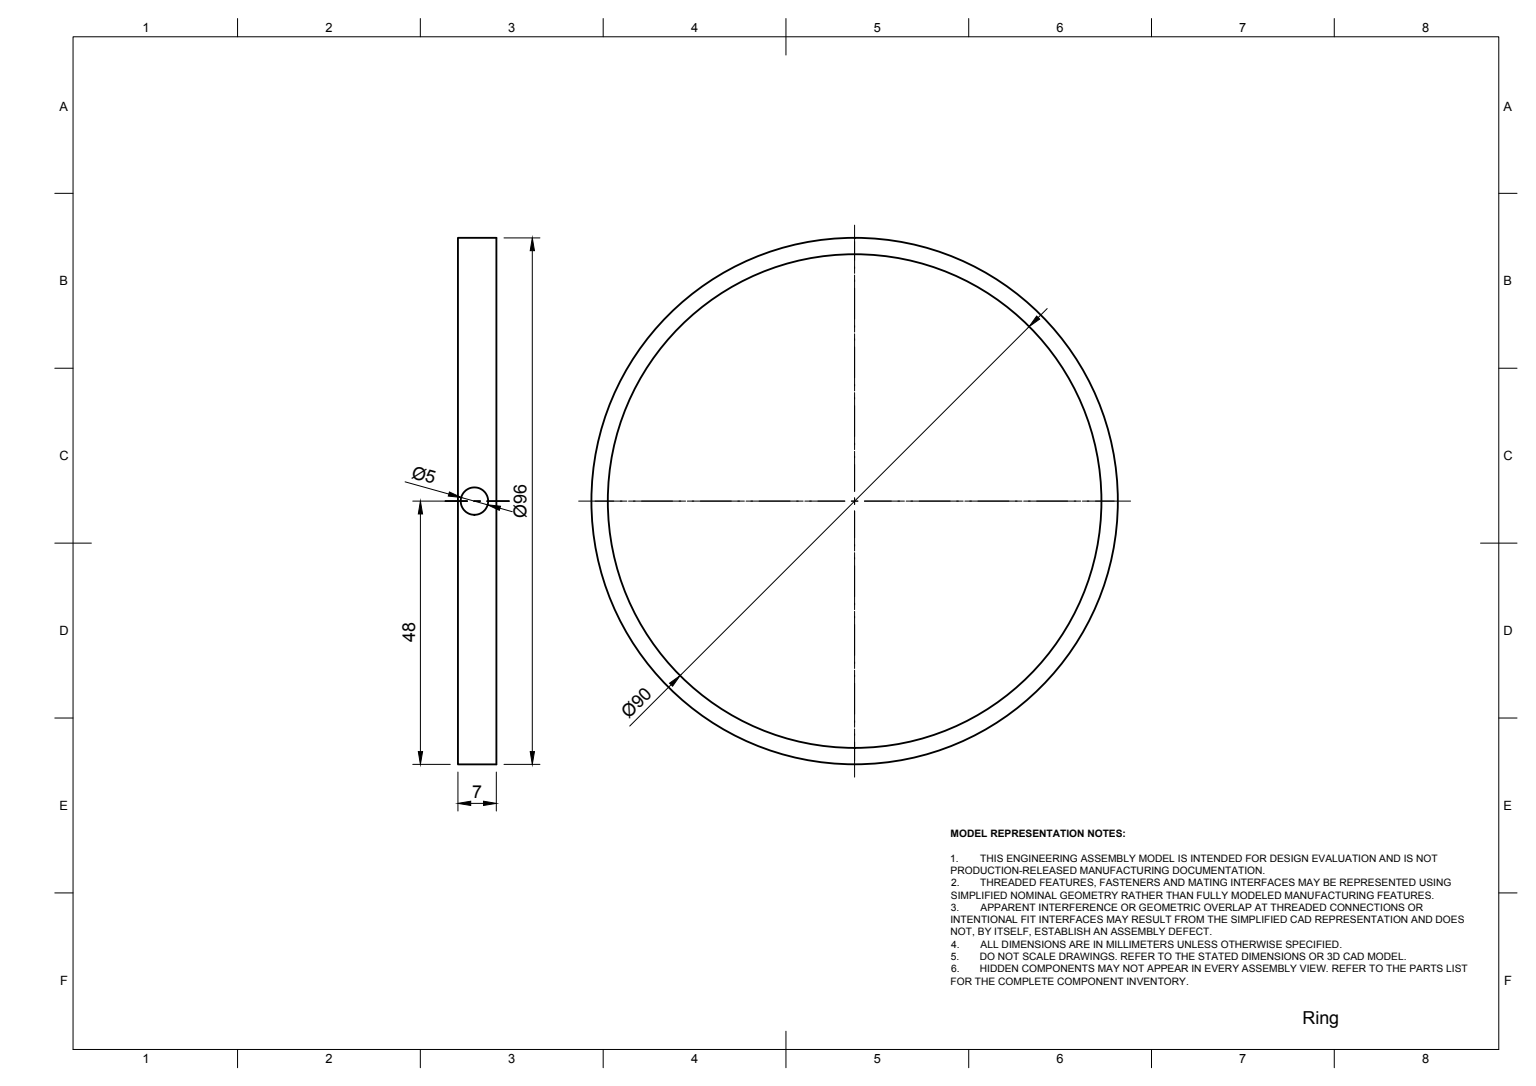
ISO-10303-21;
HEADER;
/* Generated by software containing ST-Developer
 * from STEP Tools, Inc. (www.steptools.com) 
 */

FILE_DESCRIPTION(
/* description */ (''),
/* implementation_level */ '2;1');

FILE_NAME(
/* name */ 'Ring.step',
/* time_stamp */ '2026-10-04T12:17:52-07:00',
/* author */ (''),
/* organization */ (''),
/* preprocessor_version */ 'ST-DEVELOPER v20.2',
/* originating_system */ 'Autodesk Translation Framework v15.15.0.0',
/* authorisation */ '');

FILE_SCHEMA (('AUTOMOTIVE_DESIGN { 1 0 10303 214 3 1 1 }'));
ENDSEC;

DATA;
#10=MECHANICAL_DESIGN_GEOMETRIC_PRESENTATION_REPRESENTATION('',(#65),#1602);
#43=B_SPLINE_CURVE_WITH_KNOTS('',3,(#1356,#1357,#1358,#1359,#1360,#1361,
#1362,#1363,#1364,#1365,#1366,#1367,#1368,#1369,#1370,#1371,#1372,#1373,
#1374,#1375,#1376,#1377,#1378,#1379,#1380,#1381,#1382,#1383,#1384,#1385,
#1386,#1387,#1388,#1389),.UNSPECIFIED.,.T.,.F.,(4,2,2,2,2,2,2,2,2,2,2,2,
2,2,2,2,4),(0.,0.0941899649900925,0.188379929980185,0.282569871539204,0.376759813098223,
0.470949754657242,0.565139696216261,0.659329661206353,0.753519626196446,
0.847709591186538,0.941899556176631,1.03608949773565,1.13027943929467,1.22446938085369,
1.31865932241271,1.4128492874028,1.50703925239289),.UNSPECIFIED.);
#44=B_SPLINE_CURVE_WITH_KNOTS('',3,(#1392,#1393,#1394,#1395,#1396,#1397,
#1398,#1399,#1400,#1401,#1402,#1403,#1404,#1405,#1406,#1407,#1408,#1409,
#1410,#1411,#1412,#1413,#1414,#1415,#1416,#1417,#1418,#1419,#1420,#1421,
#1422,#1423,#1424,#1425),.UNSPECIFIED.,.T.,.F.,(4,2,2,2,2,2,2,2,2,2,2,2,
2,2,2,2,4),(-1.50707960704781,-1.41288711643541,-1.318694625823,-1.22450216555443,
-1.13030970528586,-1.03611724501729,-0.941924784748718,-0.847732294136312,
-0.753539803523906,-0.6593473129115,-0.565154822299094,-0.470962362030524,
-0.376769901761953,-0.282577441493383,-0.188384981224812,-0.094192490612406,
0.),.UNSPECIFIED.);
#45=B_SPLINE_CURVE_WITH_KNOTS('',3,(#1428,#1429,#1430,#1431,#1432,#1433,
#1434,#1435,#1436,#1437,#1438,#1439,#1440,#1441,#1442,#1443,#1444,#1445,
#1446,#1447,#1448,#1449,#1450,#1451,#1452,#1453,#1454,#1455,#1456,#1457,
#1458,#1459,#1460,#1461),.UNSPECIFIED.,.T.,.F.,(4,2,2,2,2,2,2,2,2,2,2,2,
2,2,2,2,4),(-1.50707960704781,-1.41288711643541,-1.318694625823,-1.22450216555443,
-1.13030970528586,-1.03611724501729,-0.941924784748719,-0.847732294136313,
-0.753539803523906,-0.6593473129115,-0.565154822299094,-0.470962362030524,
-0.376769901761953,-0.282577441493383,-0.188384981224812,-0.0941924906124062,
0.),.UNSPECIFIED.);
#46=B_SPLINE_CURVE_WITH_KNOTS('',3,(#1464,#1465,#1466,#1467,#1468,#1469,
#1470,#1471,#1472,#1473,#1474,#1475,#1476,#1477,#1478,#1479,#1480,#1481,
#1482,#1483,#1484,#1485,#1486,#1487,#1488,#1489,#1490,#1491,#1492,#1493,
#1494,#1495,#1496,#1497),.UNSPECIFIED.,.T.,.F.,(4,2,2,2,2,2,2,2,2,2,2,2,
2,2,2,2,4),(0.,0.0941899649900927,0.188379929980185,0.282569871539204,0.376759813098223,
0.470949754657242,0.565139696216261,0.659329661206353,0.753519626196446,
0.847709591186538,0.941899556176631,1.03608949773565,1.13027943929467,1.22446938085369,
1.31865932241271,1.4128492874028,1.50703925239289),.UNSPECIFIED.);
#49=SHAPE_REPRESENTATION_RELATIONSHIP('SRR','None',#1636,#57);
#57=ADVANCED_BREP_SHAPE_REPRESENTATION('',(#73),#1596);
#65=STYLED_ITEM('',(#1684),#73);
#73=MANIFOLD_SOLID_BREP('Body1',#776);
#81=FACE_BOUND('',#230,.T.);
#82=FACE_BOUND('',#231,.T.);
#83=FACE_BOUND('',#233,.T.);
#84=FACE_BOUND('',#234,.T.);
#85=FACE_BOUND('',#236,.T.);
#86=FACE_BOUND('',#238,.T.);
#113=CIRCLE('',#921,45.);
#114=CIRCLE('',#922,45.);
#115=CIRCLE('',#924,48.);
#116=CIRCLE('',#925,48.);
#143=CYLINDRICAL_SURFACE('',#918,2.5);
#144=CYLINDRICAL_SURFACE('',#919,2.5);
#145=CYLINDRICAL_SURFACE('',#920,45.);
#146=CYLINDRICAL_SURFACE('',#923,48.);
#178=FACE_OUTER_BOUND('',#227,.T.);
#179=FACE_OUTER_BOUND('',#228,.T.);
#180=FACE_OUTER_BOUND('',#229,.T.);
#181=FACE_OUTER_BOUND('',#232,.T.);
#182=FACE_OUTER_BOUND('',#235,.T.);
#183=FACE_OUTER_BOUND('',#237,.T.);
#227=EDGE_LOOP('',(#630,#631,#632,#633));
#228=EDGE_LOOP('',(#634,#635,#636,#637));
#229=EDGE_LOOP('',(#638,#639,#640,#641));
#230=EDGE_LOOP('',(#642));
#231=EDGE_LOOP('',(#643));
#232=EDGE_LOOP('',(#644,#645,#646,#647));
#233=EDGE_LOOP('',(#648));
#234=EDGE_LOOP('',(#649));
#235=EDGE_LOOP('',(#650));
#236=EDGE_LOOP('',(#651));
#237=EDGE_LOOP('',(#652));
#238=EDGE_LOOP('',(#653));
#300=LINE('',#1391,#349);
#301=LINE('',#1463,#350);
#302=LINE('',#1502,#351);
#303=LINE('',#1508,#352);
#349=VECTOR('',#1108,2.5);
#350=VECTOR('',#1111,2.5);
#351=VECTOR('',#1116,45.);
#352=VECTOR('',#1123,48.);
#399=VERTEX_POINT('',#1355);
#400=VERTEX_POINT('',#1390);
#401=VERTEX_POINT('',#1427);
#402=VERTEX_POINT('',#1462);
#403=VERTEX_POINT('',#1499);
#404=VERTEX_POINT('',#1501);
#405=VERTEX_POINT('',#1505);
#406=VERTEX_POINT('',#1507);
#480=EDGE_CURVE('',#399,#399,#43,.T.);
#481=EDGE_CURVE('',#399,#400,#300,.T.);
#482=EDGE_CURVE('',#400,#400,#44,.T.);
#483=EDGE_CURVE('',#401,#401,#45,.T.);
#484=EDGE_CURVE('',#401,#402,#301,.T.);
#485=EDGE_CURVE('',#402,#402,#46,.T.);
#486=EDGE_CURVE('',#403,#403,#113,.T.);
#487=EDGE_CURVE('',#403,#404,#302,.T.);
#488=EDGE_CURVE('',#404,#404,#114,.T.);
#489=EDGE_CURVE('',#405,#405,#115,.T.);
#490=EDGE_CURVE('',#405,#406,#303,.T.);
#491=EDGE_CURVE('',#406,#406,#116,.T.);
#630=ORIENTED_EDGE('',*,*,#480,.F.);
#631=ORIENTED_EDGE('',*,*,#481,.T.);
#632=ORIENTED_EDGE('',*,*,#482,.F.);
#633=ORIENTED_EDGE('',*,*,#481,.F.);
#634=ORIENTED_EDGE('',*,*,#483,.F.);
#635=ORIENTED_EDGE('',*,*,#484,.T.);
#636=ORIENTED_EDGE('',*,*,#485,.F.);
#637=ORIENTED_EDGE('',*,*,#484,.F.);
#638=ORIENTED_EDGE('',*,*,#486,.T.);
#639=ORIENTED_EDGE('',*,*,#487,.T.);
#640=ORIENTED_EDGE('',*,*,#488,.F.);
#641=ORIENTED_EDGE('',*,*,#487,.F.);
#642=ORIENTED_EDGE('',*,*,#482,.T.);
#643=ORIENTED_EDGE('',*,*,#483,.T.);
#644=ORIENTED_EDGE('',*,*,#489,.F.);
#645=ORIENTED_EDGE('',*,*,#490,.T.);
#646=ORIENTED_EDGE('',*,*,#491,.T.);
#647=ORIENTED_EDGE('',*,*,#490,.F.);
#648=ORIENTED_EDGE('',*,*,#480,.T.);
#649=ORIENTED_EDGE('',*,*,#485,.T.);
#650=ORIENTED_EDGE('',*,*,#489,.T.);
#651=ORIENTED_EDGE('',*,*,#488,.T.);
#652=ORIENTED_EDGE('',*,*,#491,.F.);
#653=ORIENTED_EDGE('',*,*,#486,.F.);
#715=PLANE('',#926);
#716=PLANE('',#927);
#750=ADVANCED_FACE('',(#178),#143,.F.);
#751=ADVANCED_FACE('',(#179),#144,.F.);
#752=ADVANCED_FACE('',(#180,#81,#82),#145,.F.);
#753=ADVANCED_FACE('',(#181,#83,#84),#146,.T.);
#754=ADVANCED_FACE('',(#182,#85),#715,.T.);
#755=ADVANCED_FACE('',(#183,#86),#716,.F.);
#776=CLOSED_SHELL('',(#750,#751,#752,#753,#754,#755));
#917=AXIS2_PLACEMENT_3D('',#1353,#1104,#1105);
#918=AXIS2_PLACEMENT_3D('',#1354,#1106,#1107);
#919=AXIS2_PLACEMENT_3D('',#1426,#1109,#1110);
#920=AXIS2_PLACEMENT_3D('',#1498,#1112,#1113);
#921=AXIS2_PLACEMENT_3D('',#1500,#1114,#1115);
#922=AXIS2_PLACEMENT_3D('',#1503,#1117,#1118);
#923=AXIS2_PLACEMENT_3D('',#1504,#1119,#1120);
#924=AXIS2_PLACEMENT_3D('',#1506,#1121,#1122);
#925=AXIS2_PLACEMENT_3D('',#1509,#1124,#1125);
#926=AXIS2_PLACEMENT_3D('',#1510,#1126,#1127);
#927=AXIS2_PLACEMENT_3D('',#1511,#1128,#1129);
#1104=DIRECTION('axis',(0.,0.,1.));
#1105=DIRECTION('refdir',(1.,0.,0.));
#1106=DIRECTION('center_axis',(0.,0.,1.));
#1107=DIRECTION('ref_axis',(1.,0.,0.));
#1108=DIRECTION('',(0.,0.,1.));
#1109=DIRECTION('center_axis',(0.,0.,1.));
#1110=DIRECTION('ref_axis',(1.,0.,0.));
#1111=DIRECTION('',(0.,0.,1.));
#1112=DIRECTION('center_axis',(0.,-1.,0.));
#1113=DIRECTION('ref_axis',(1.,0.,0.));
#1114=DIRECTION('center_axis',(0.,1.,0.));
#1115=DIRECTION('ref_axis',(1.,0.,0.));
#1116=DIRECTION('',(0.,-1.,0.));
#1117=DIRECTION('center_axis',(0.,1.,0.));
#1118=DIRECTION('ref_axis',(1.,0.,0.));
#1119=DIRECTION('center_axis',(0.,-1.,0.));
#1120=DIRECTION('ref_axis',(1.,0.,0.));
#1121=DIRECTION('center_axis',(0.,-1.,0.));
#1122=DIRECTION('ref_axis',(1.,0.,0.));
#1123=DIRECTION('',(0.,1.,0.));
#1124=DIRECTION('center_axis',(0.,-1.,0.));
#1125=DIRECTION('ref_axis',(1.,0.,0.));
#1126=DIRECTION('center_axis',(0.,-1.,0.));
#1127=DIRECTION('ref_axis',(1.,0.,0.));
#1128=DIRECTION('center_axis',(0.,-1.,0.));
#1129=DIRECTION('ref_axis',(1.,0.,0.));
#1353=CARTESIAN_POINT('',(0.,0.,0.));
#1354=CARTESIAN_POINT('Origin',(0.,0.,0.));
#1355=CARTESIAN_POINT('',(-2.5,-6.93889390390723E-17,2.06514837824155));
#1356=CARTESIAN_POINT('Ctrl Pts',(-2.5,0.,2.06514837824153));
#1357=CARTESIAN_POINT('Ctrl Pts',(-2.5,-0.313966549966975,2.06514837824153));
#1358=CARTESIAN_POINT('Ctrl Pts',(-2.43724208175823,-0.648821661237632,
2.06174633522331));
#1359=CARTESIAN_POINT('Ctrl Pts',(-2.18209026124743,-1.26475318832061,2.04945469062714));
#1360=CARTESIAN_POINT('Ctrl Pts',(-1.98969948627882,-1.54583441965392,2.04074211479646));
#1361=CARTESIAN_POINT('Ctrl Pts',(-1.54583447486274,-1.98969943106999,2.02438414468301));
#1362=CARTESIAN_POINT('Ctrl Pts',(-1.26475321841524,-2.18209024745813,2.0156767273781));
#1363=CARTESIAN_POINT('Ctrl Pts',(-0.648821611717717,-2.43724210359452,
2.00339687904366));
#1364=CARTESIAN_POINT('Ctrl Pts',(-0.313966471863397,-2.5,1.99999999999999));
#1365=CARTESIAN_POINT('Ctrl Pts',(0.313966471863396,-2.5,1.99999999999999));
#1366=CARTESIAN_POINT('Ctrl Pts',(0.648821611717716,-2.43724210359452,2.00339687904366));
#1367=CARTESIAN_POINT('Ctrl Pts',(1.26475321841524,-2.18209024745813,2.0156767273781));
#1368=CARTESIAN_POINT('Ctrl Pts',(1.54583447486274,-1.98969943106999,2.02438414468301));
#1369=CARTESIAN_POINT('Ctrl Pts',(1.98969948627882,-1.54583441965392,2.04074211479646));
#1370=CARTESIAN_POINT('Ctrl Pts',(2.18209026124743,-1.26475318832061,2.04945469062714));
#1371=CARTESIAN_POINT('Ctrl Pts',(2.43724208175823,-0.648821661237632,2.06174633522331));
#1372=CARTESIAN_POINT('Ctrl Pts',(2.5,-0.313966549966975,2.06514837824153));
#1373=CARTESIAN_POINT('Ctrl Pts',(2.5,0.313966549966975,2.06514837824153));
#1374=CARTESIAN_POINT('Ctrl Pts',(2.43724208175823,0.648821661237632,2.06174633522331));
#1375=CARTESIAN_POINT('Ctrl Pts',(2.18209026124743,1.26475318832061,2.04945469062714));
#1376=CARTESIAN_POINT('Ctrl Pts',(1.98969948627882,1.54583441965392,2.04074211479646));
#1377=CARTESIAN_POINT('Ctrl Pts',(1.54583447486274,1.98969943106999,2.02438414468301));
#1378=CARTESIAN_POINT('Ctrl Pts',(1.26475321841524,2.18209024745813,2.0156767273781));
#1379=CARTESIAN_POINT('Ctrl Pts',(0.648821611717718,2.43724210359452,2.00339687904366));
#1380=CARTESIAN_POINT('Ctrl Pts',(0.313966471863397,2.5,1.99999999999999));
#1381=CARTESIAN_POINT('Ctrl Pts',(-0.313966471863395,2.5,1.99999999999999));
#1382=CARTESIAN_POINT('Ctrl Pts',(-0.648821611717715,2.43724210359452,2.00339687904366));
#1383=CARTESIAN_POINT('Ctrl Pts',(-1.26475321841524,2.18209024745813,2.0156767273781));
#1384=CARTESIAN_POINT('Ctrl Pts',(-1.54583447486274,1.98969943107,2.02438414468301));
#1385=CARTESIAN_POINT('Ctrl Pts',(-1.98969948627882,1.54583441965392,2.04074211479646));
#1386=CARTESIAN_POINT('Ctrl Pts',(-2.18209026124743,1.26475318832061,2.04945469062714));
#1387=CARTESIAN_POINT('Ctrl Pts',(-2.43724208175823,0.648821661237633,2.06174633522331));
#1388=CARTESIAN_POINT('Ctrl Pts',(-2.5,0.313966549966975,2.06514837824153));
#1389=CARTESIAN_POINT('Ctrl Pts',(-2.5,-1.38777878078145E-16,2.06514837824153));
#1390=CARTESIAN_POINT('',(-2.5,-1.38777878078145E-16,5.06949811097144));
#1391=CARTESIAN_POINT('',(-2.5,-3.06161699786838E-16,0.));
#1392=CARTESIAN_POINT('Ctrl Pts',(-2.5,-2.08166817117217E-16,5.06949811097143));
#1393=CARTESIAN_POINT('Ctrl Pts',(-2.5,0.31397496870802,5.06949811097143));
#1394=CARTESIAN_POINT('Ctrl Pts',(-2.43723879407712,0.648833697924306,5.06586836285142));
#1395=CARTESIAN_POINT('Ctrl Pts',(-2.18208453863604,1.26476290215938,5.05275507922167));
#1396=CARTESIAN_POINT('Ctrl Pts',(-1.98969504628277,1.54583885964997,5.04346052213127));
#1397=CARTESIAN_POINT('Ctrl Pts',(-1.54583893114345,1.98969497478929,5.02601073765469));
#1398=CARTESIAN_POINT('Ctrl Pts',(-1.26476294130742,2.18208452114785,5.01672244237508));
#1399=CARTESIAN_POINT('Ctrl Pts',(-0.64883363366083,2.4372388219696,5.00362347878181));
#1400=CARTESIAN_POINT('Ctrl Pts',(-0.313974867561901,2.5,5.));
#1401=CARTESIAN_POINT('Ctrl Pts',(0.313974867561902,2.5,5.));
#1402=CARTESIAN_POINT('Ctrl Pts',(0.648833633660831,2.4372388219696,5.00362347878181));
#1403=CARTESIAN_POINT('Ctrl Pts',(1.26476294130743,2.18208452114784,5.01672244237508));
#1404=CARTESIAN_POINT('Ctrl Pts',(1.54583893114345,1.98969497478929,5.02601073765469));
#1405=CARTESIAN_POINT('Ctrl Pts',(1.98969504628277,1.54583885964996,5.04346052213127));
#1406=CARTESIAN_POINT('Ctrl Pts',(2.18208453863604,1.26476290215938,5.05275507922167));
#1407=CARTESIAN_POINT('Ctrl Pts',(2.43723879407712,0.648833697924305,5.06586836285142));
#1408=CARTESIAN_POINT('Ctrl Pts',(2.5,0.31397496870802,5.06949811097143));
#1409=CARTESIAN_POINT('Ctrl Pts',(2.5,-0.31397496870802,5.06949811097143));
#1410=CARTESIAN_POINT('Ctrl Pts',(2.43723879407712,-0.648833697924305,5.06586836285142));
#1411=CARTESIAN_POINT('Ctrl Pts',(2.18208453863604,-1.26476290215938,5.05275507922167));
#1412=CARTESIAN_POINT('Ctrl Pts',(1.98969504628277,-1.54583885964996,5.04346052213127));
#1413=CARTESIAN_POINT('Ctrl Pts',(1.54583893114345,-1.98969497478929,5.02601073765469));
#1414=CARTESIAN_POINT('Ctrl Pts',(1.26476294130743,-2.18208452114784,5.01672244237508));
#1415=CARTESIAN_POINT('Ctrl Pts',(0.648833633660831,-2.4372388219696,5.00362347878181));
#1416=CARTESIAN_POINT('Ctrl Pts',(0.313974867561901,-2.5,5.));
#1417=CARTESIAN_POINT('Ctrl Pts',(-0.313974867561902,-2.5,5.));
#1418=CARTESIAN_POINT('Ctrl Pts',(-0.648833633660832,-2.4372388219696,5.00362347878181));
#1419=CARTESIAN_POINT('Ctrl Pts',(-1.26476294130743,-2.18208452114784,5.01672244237508));
#1420=CARTESIAN_POINT('Ctrl Pts',(-1.54583893114345,-1.98969497478929,5.02601073765469));
#1421=CARTESIAN_POINT('Ctrl Pts',(-1.98969504628277,-1.54583885964996,5.04346052213127));
#1422=CARTESIAN_POINT('Ctrl Pts',(-2.18208453863604,-1.26476290215938,5.05275507922167));
#1423=CARTESIAN_POINT('Ctrl Pts',(-2.43723879407712,-0.648833697924305,
5.06586836285142));
#1424=CARTESIAN_POINT('Ctrl Pts',(-2.5,-0.31397496870802,5.06949811097143));
#1425=CARTESIAN_POINT('Ctrl Pts',(-2.5,6.93889390390723E-17,5.06949811097143));
#1426=CARTESIAN_POINT('Origin',(0.,0.,96.6));
#1427=CARTESIAN_POINT('',(-2.5,6.93889390390723E-17,94.9305018890286));
#1428=CARTESIAN_POINT('Ctrl Pts',(-2.5,1.38777878078145E-16,94.9305018890286));
#1429=CARTESIAN_POINT('Ctrl Pts',(-2.5,-0.31397496870802,94.9305018890286));
#1430=CARTESIAN_POINT('Ctrl Pts',(-2.43723879407712,-0.648833697924305,
94.9341316371486));
#1431=CARTESIAN_POINT('Ctrl Pts',(-2.18208453863604,-1.26476290215938,94.9472449207783));
#1432=CARTESIAN_POINT('Ctrl Pts',(-1.98969504628277,-1.54583885964996,94.9565394778687));
#1433=CARTESIAN_POINT('Ctrl Pts',(-1.54583893114345,-1.98969497478929,94.9739892623453));
#1434=CARTESIAN_POINT('Ctrl Pts',(-1.26476294130743,-2.18208452114784,94.9832775576249));
#1435=CARTESIAN_POINT('Ctrl Pts',(-0.648833633660833,-2.4372388219696,94.9963765212182));
#1436=CARTESIAN_POINT('Ctrl Pts',(-0.313974867561903,-2.5,95.));
#1437=CARTESIAN_POINT('Ctrl Pts',(0.313974867561902,-2.5,95.));
#1438=CARTESIAN_POINT('Ctrl Pts',(0.648833633660832,-2.4372388219696,94.9963765212182));
#1439=CARTESIAN_POINT('Ctrl Pts',(1.26476294130743,-2.18208452114784,94.9832775576249));
#1440=CARTESIAN_POINT('Ctrl Pts',(1.54583893114345,-1.98969497478929,94.9739892623453));
#1441=CARTESIAN_POINT('Ctrl Pts',(1.98969504628277,-1.54583885964996,94.9565394778687));
#1442=CARTESIAN_POINT('Ctrl Pts',(2.18208453863604,-1.26476290215938,94.9472449207783));
#1443=CARTESIAN_POINT('Ctrl Pts',(2.43723879407712,-0.648833697924305,94.9341316371486));
#1444=CARTESIAN_POINT('Ctrl Pts',(2.5,-0.31397496870802,94.9305018890286));
#1445=CARTESIAN_POINT('Ctrl Pts',(2.5,0.31397496870802,94.9305018890286));
#1446=CARTESIAN_POINT('Ctrl Pts',(2.43723879407712,0.648833697924305,94.9341316371486));
#1447=CARTESIAN_POINT('Ctrl Pts',(2.18208453863604,1.26476290215938,94.9472449207783));
#1448=CARTESIAN_POINT('Ctrl Pts',(1.98969504628277,1.54583885964996,94.9565394778687));
#1449=CARTESIAN_POINT('Ctrl Pts',(1.54583893114345,1.98969497478929,94.9739892623453));
#1450=CARTESIAN_POINT('Ctrl Pts',(1.26476294130743,2.18208452114784,94.9832775576249));
#1451=CARTESIAN_POINT('Ctrl Pts',(0.648833633660832,2.4372388219696,94.9963765212182));
#1452=CARTESIAN_POINT('Ctrl Pts',(0.313974867561903,2.5,95.));
#1453=CARTESIAN_POINT('Ctrl Pts',(-0.313974867561901,2.5,95.));
#1454=CARTESIAN_POINT('Ctrl Pts',(-0.648833633660831,2.4372388219696,94.9963765212182));
#1455=CARTESIAN_POINT('Ctrl Pts',(-1.26476294130743,2.18208452114784,94.9832775576249));
#1456=CARTESIAN_POINT('Ctrl Pts',(-1.54583893114345,1.98969497478929,94.9739892623453));
#1457=CARTESIAN_POINT('Ctrl Pts',(-1.98969504628277,1.54583885964997,94.9565394778687));
#1458=CARTESIAN_POINT('Ctrl Pts',(-2.18208453863604,1.26476290215938,94.9472449207783));
#1459=CARTESIAN_POINT('Ctrl Pts',(-2.43723879407712,0.648833697924306,94.9341316371486));
#1460=CARTESIAN_POINT('Ctrl Pts',(-2.5,0.313974968708021,94.9305018890286));
#1461=CARTESIAN_POINT('Ctrl Pts',(-2.5,0.,94.9305018890286));
#1462=CARTESIAN_POINT('',(-2.5,-1.38777878078145E-16,97.9348516217584));
#1463=CARTESIAN_POINT('',(-2.5,-3.06161699786838E-16,96.6));
#1464=CARTESIAN_POINT('Ctrl Pts',(-2.5,0.,97.9348516217585));
#1465=CARTESIAN_POINT('Ctrl Pts',(-2.5,0.313966549966976,97.9348516217585));
#1466=CARTESIAN_POINT('Ctrl Pts',(-2.43724208175823,0.648821661237634,97.9382536647767));
#1467=CARTESIAN_POINT('Ctrl Pts',(-2.18209026124743,1.26475318832061,97.9505453093728));
#1468=CARTESIAN_POINT('Ctrl Pts',(-1.98969948627882,1.54583441965392,97.9592578852035));
#1469=CARTESIAN_POINT('Ctrl Pts',(-1.54583447486274,1.98969943107,97.975615855317));
#1470=CARTESIAN_POINT('Ctrl Pts',(-1.26475321841524,2.18209024745813,97.9843232726219));
#1471=CARTESIAN_POINT('Ctrl Pts',(-0.648821611717716,2.43724210359452,97.9966031209564));
#1472=CARTESIAN_POINT('Ctrl Pts',(-0.313966471863395,2.5,98.));
#1473=CARTESIAN_POINT('Ctrl Pts',(0.313966471863397,2.5,98.));
#1474=CARTESIAN_POINT('Ctrl Pts',(0.648821611717718,2.43724210359452,97.9966031209564));
#1475=CARTESIAN_POINT('Ctrl Pts',(1.26475321841524,2.18209024745813,97.9843232726219));
#1476=CARTESIAN_POINT('Ctrl Pts',(1.54583447486274,1.98969943106999,97.975615855317));
#1477=CARTESIAN_POINT('Ctrl Pts',(1.98969948627882,1.54583441965392,97.9592578852035));
#1478=CARTESIAN_POINT('Ctrl Pts',(2.18209026124743,1.26475318832061,97.9505453093728));
#1479=CARTESIAN_POINT('Ctrl Pts',(2.43724208175823,0.648821661237632,97.9382536647767));
#1480=CARTESIAN_POINT('Ctrl Pts',(2.5,0.313966549966975,97.9348516217585));
#1481=CARTESIAN_POINT('Ctrl Pts',(2.5,-0.313966549966975,97.9348516217585));
#1482=CARTESIAN_POINT('Ctrl Pts',(2.43724208175823,-0.648821661237632,97.9382536647767));
#1483=CARTESIAN_POINT('Ctrl Pts',(2.18209026124743,-1.26475318832061,97.9505453093728));
#1484=CARTESIAN_POINT('Ctrl Pts',(1.98969948627882,-1.54583441965392,97.9592578852035));
#1485=CARTESIAN_POINT('Ctrl Pts',(1.54583447486274,-1.98969943106999,97.975615855317));
#1486=CARTESIAN_POINT('Ctrl Pts',(1.26475321841524,-2.18209024745813,97.9843232726219));
#1487=CARTESIAN_POINT('Ctrl Pts',(0.648821611717717,-2.43724210359452,97.9966031209564));
#1488=CARTESIAN_POINT('Ctrl Pts',(0.313966471863396,-2.5,98.));
#1489=CARTESIAN_POINT('Ctrl Pts',(-0.313966471863397,-2.5,98.));
#1490=CARTESIAN_POINT('Ctrl Pts',(-0.648821611717717,-2.43724210359452,
97.9966031209564));
#1491=CARTESIAN_POINT('Ctrl Pts',(-1.26475321841524,-2.18209024745813,97.9843232726219));
#1492=CARTESIAN_POINT('Ctrl Pts',(-1.54583447486274,-1.98969943106999,97.975615855317));
#1493=CARTESIAN_POINT('Ctrl Pts',(-1.98969948627882,-1.54583441965392,97.9592578852035));
#1494=CARTESIAN_POINT('Ctrl Pts',(-2.18209026124743,-1.26475318832061,97.9505453093728));
#1495=CARTESIAN_POINT('Ctrl Pts',(-2.43724208175823,-0.648821661237633,
97.9382536647767));
#1496=CARTESIAN_POINT('Ctrl Pts',(-2.5,-0.313966549966975,97.9348516217585));
#1497=CARTESIAN_POINT('Ctrl Pts',(-2.5,1.38777878078145E-16,97.9348516217585));
#1498=CARTESIAN_POINT('Origin',(0.,4.,50.));
#1499=CARTESIAN_POINT('',(-45.,4.,50.));
#1500=CARTESIAN_POINT('Origin',(0.,4.,50.));
#1501=CARTESIAN_POINT('',(-45.,-3.,50.));
#1502=CARTESIAN_POINT('',(-45.,4.,50.));
#1503=CARTESIAN_POINT('Origin',(0.,-3.,50.));
#1504=CARTESIAN_POINT('Origin',(0.,4.,50.));
#1505=CARTESIAN_POINT('',(-48.,-3.,50.));
#1506=CARTESIAN_POINT('Origin',(0.,-3.,50.));
#1507=CARTESIAN_POINT('',(-48.,4.,50.));
#1508=CARTESIAN_POINT('',(-48.,4.,50.));
#1509=CARTESIAN_POINT('Origin',(0.,4.,50.));
#1510=CARTESIAN_POINT('Origin',(0.,-3.,50.));
#1511=CARTESIAN_POINT('Origin',(0.,4.,50.));
#1586=UNCERTAINTY_MEASURE_WITH_UNIT(LENGTH_MEASURE(0.01),#1603,
'DISTANCE_ACCURACY_VALUE',
'Maximum model space distance between geometric entities at asserted c
onnectivities');
#1592=UNCERTAINTY_MEASURE_WITH_UNIT(LENGTH_MEASURE(0.01),#1603,
'DISTANCE_ACCURACY_VALUE',
'Maximum model space distance between geometric entities at asserted c
onnectivities');
#1596=(
GEOMETRIC_REPRESENTATION_CONTEXT(3)
GLOBAL_UNCERTAINTY_ASSIGNED_CONTEXT((#1586))
GLOBAL_UNIT_ASSIGNED_CONTEXT((#1603,#1605,#1606))
REPRESENTATION_CONTEXT('','3D')
);
#1602=(
GEOMETRIC_REPRESENTATION_CONTEXT(3)
GLOBAL_UNCERTAINTY_ASSIGNED_CONTEXT((#1592))
GLOBAL_UNIT_ASSIGNED_CONTEXT((#1603,#1605,#1606))
REPRESENTATION_CONTEXT('','3D')
);
#1603=(
LENGTH_UNIT()
NAMED_UNIT(*)
SI_UNIT(.MILLI.,.METRE.)
);
#1605=(
NAMED_UNIT(*)
PLANE_ANGLE_UNIT()
SI_UNIT($,.RADIAN.)
);
#1606=(
NAMED_UNIT(*)
SI_UNIT($,.STERADIAN.)
SOLID_ANGLE_UNIT()
);
#1610=SHAPE_DEFINITION_REPRESENTATION(#1619,#1636);
#1619=PRODUCT_DEFINITION_SHAPE('',$,#1646);
#1636=SHAPE_REPRESENTATION('',(#917),#1596);
#1642=PRODUCT_DEFINITION_CONTEXT('part definition',#1671,'design');
#1646=PRODUCT_DEFINITION('Ring','Ring',#1655,#1642);
#1655=PRODUCT_DEFINITION_FORMATION('',$,#1676);
#1671=APPLICATION_CONTEXT(
'Core Data for Automotive Mechanical Design Process');
#1672=PRODUCT_CONTEXT('part definition',#1671,'mechanical');
#1676=PRODUCT('Ring','Ring',$,(#1672));
#1684=PRESENTATION_STYLE_ASSIGNMENT((#1688));
#1688=SURFACE_STYLE_USAGE(.BOTH.,#1692);
#1692=SURFACE_SIDE_STYLE('',(#1696));
#1696=SURFACE_STYLE_FILL_AREA(#1700);
#1700=FILL_AREA_STYLE('Opaque(160,160,160)',(#1704));
#1704=FILL_AREA_STYLE_COLOUR('Opaque(160,160,160)',#1708);
#1708=COLOUR_RGB('Opaque(160,160,160)', 0.66274510, 0.83137255, 0.94901961);
ENDSEC;
END-ISO-10303-21;
